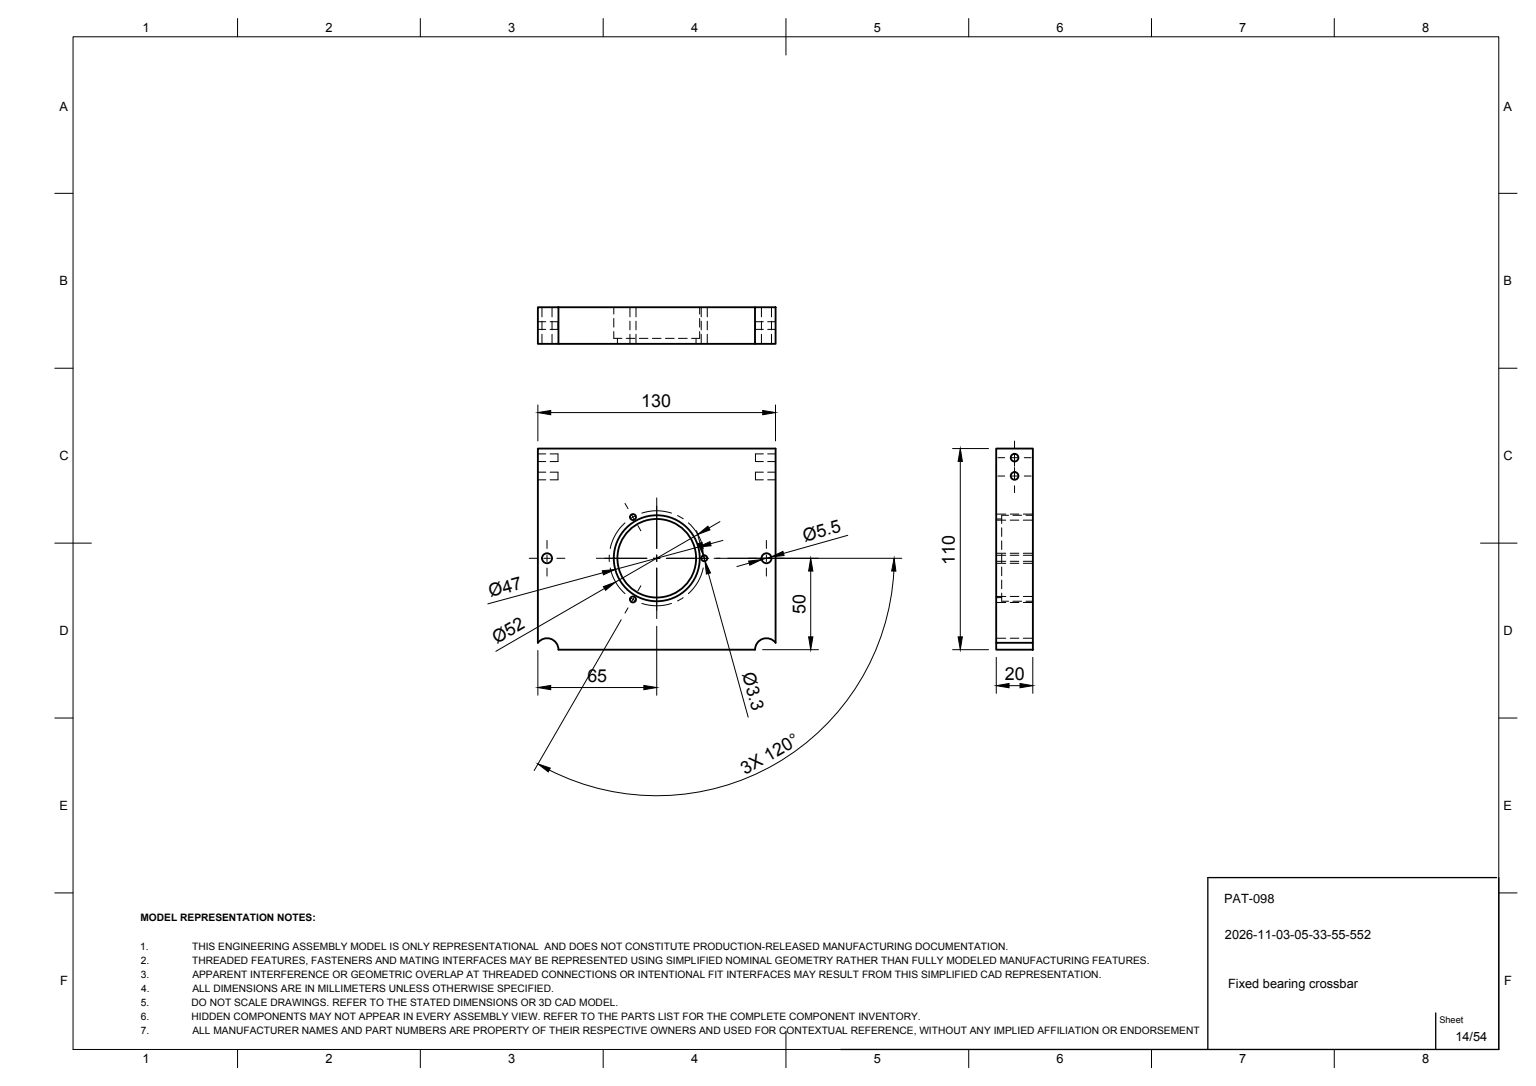
ISO-10303-21;
HEADER;
/* Generated by software containing ST-Developer
 * from STEP Tools, Inc. (www.steptools.com) 
 */

FILE_DESCRIPTION(
/* description */ ('Spring compression tester'),
/* implementation_level */ '2;1');

FILE_NAME(
/* name */ 'Fixed bearing crossbar.step',
/* time_stamp */ '2026-10-28T03:24:11-07:00',
/* author */ (''),
/* organization */ (''),
/* preprocessor_version */ 'ST-DEVELOPER v20.2',
/* originating_system */ 'Autodesk Translation Framework v15.17.0.0',
/* authorisation */ '');

FILE_SCHEMA (('AUTOMOTIVE_DESIGN { 1 0 10303 214 3 1 1 }'));
ENDSEC;

DATA;
#10=MECHANICAL_DESIGN_GEOMETRIC_PRESENTATION_REPRESENTATION('',(#1115),#43521);
#995=SHAPE_REPRESENTATION_RELATIONSHIP('SRR','None',#43807,#1055);
#1055=ADVANCED_BREP_SHAPE_REPRESENTATION('',(#1190),#43467);
#1115=STYLED_ITEM('',(#44202),#1190);
#1190=MANIFOLD_SOLID_BREP('Body1',#18552);
#1359=FACE_BOUND('',#3516,.T.);
#1360=FACE_BOUND('',#3521,.T.);
#1361=FACE_BOUND('',#3522,.T.);
#1362=FACE_BOUND('',#3524,.T.);
#1363=FACE_BOUND('',#3525,.T.);
#1364=FACE_BOUND('',#3526,.T.);
#1365=FACE_BOUND('',#3527,.T.);
#1366=FACE_BOUND('',#3528,.T.);
#1367=FACE_BOUND('',#3529,.T.);
#1368=FACE_BOUND('',#3533,.T.);
#1369=FACE_BOUND('',#3534,.T.);
#1370=FACE_BOUND('',#3536,.T.);
#1371=FACE_BOUND('',#3537,.T.);
#1372=FACE_BOUND('',#3538,.T.);
#1373=FACE_BOUND('',#3539,.T.);
#1374=FACE_BOUND('',#3540,.T.);
#1375=FACE_BOUND('',#3541,.T.);
#1693=PLANE('',#19632);
#1694=PLANE('',#19636);
#1695=PLANE('',#19640);
#1696=PLANE('',#19644);
#1697=PLANE('',#19648);
#1698=PLANE('',#19658);
#1699=PLANE('',#19659);
#1700=PLANE('',#19660);
#1701=PLANE('',#19661);
#1702=PLANE('',#19662);
#1703=PLANE('',#19663);
#2342=FACE_OUTER_BOUND('',#3501,.T.);
#2343=FACE_OUTER_BOUND('',#3502,.T.);
#2344=FACE_OUTER_BOUND('',#3503,.T.);
#2345=FACE_OUTER_BOUND('',#3504,.T.);
#2346=FACE_OUTER_BOUND('',#3505,.T.);
#2347=FACE_OUTER_BOUND('',#3506,.T.);
#2348=FACE_OUTER_BOUND('',#3507,.T.);
#2349=FACE_OUTER_BOUND('',#3508,.T.);
#2350=FACE_OUTER_BOUND('',#3509,.T.);
#2351=FACE_OUTER_BOUND('',#3510,.T.);
#2352=FACE_OUTER_BOUND('',#3511,.T.);
#2353=FACE_OUTER_BOUND('',#3512,.T.);
#2354=FACE_OUTER_BOUND('',#3513,.T.);
#2355=FACE_OUTER_BOUND('',#3514,.T.);
#2356=FACE_OUTER_BOUND('',#3515,.T.);
#2357=FACE_OUTER_BOUND('',#3517,.T.);
#2358=FACE_OUTER_BOUND('',#3518,.T.);
#2359=FACE_OUTER_BOUND('',#3519,.T.);
#2360=FACE_OUTER_BOUND('',#3520,.T.);
#2361=FACE_OUTER_BOUND('',#3523,.T.);
#2362=FACE_OUTER_BOUND('',#3530,.T.);
#2363=FACE_OUTER_BOUND('',#3531,.T.);
#2364=FACE_OUTER_BOUND('',#3532,.T.);
#2365=FACE_OUTER_BOUND('',#3535,.T.);
#3501=EDGE_LOOP('',(#13009,#13010,#13011,#13012));
#3502=EDGE_LOOP('',(#13013,#13014,#13015,#13016));
#3503=EDGE_LOOP('',(#13017,#13018,#13019,#13020));
#3504=EDGE_LOOP('',(#13021,#13022,#13023,#13024));
#3505=EDGE_LOOP('',(#13025,#13026,#13027,#13028));
#3506=EDGE_LOOP('',(#13029,#13030,#13031,#13032));
#3507=EDGE_LOOP('',(#13033));
#3508=EDGE_LOOP('',(#13034,#13035,#13036,#13037));
#3509=EDGE_LOOP('',(#13038));
#3510=EDGE_LOOP('',(#13039,#13040,#13041,#13042));
#3511=EDGE_LOOP('',(#13043));
#3512=EDGE_LOOP('',(#13044,#13045,#13046,#13047));
#3513=EDGE_LOOP('',(#13048));
#3514=EDGE_LOOP('',(#13049,#13050,#13051,#13052));
#3515=EDGE_LOOP('',(#13053));
#3516=EDGE_LOOP('',(#13054));
#3517=EDGE_LOOP('',(#13055,#13056,#13057,#13058));
#3518=EDGE_LOOP('',(#13059,#13060,#13061,#13062));
#3519=EDGE_LOOP('',(#13063,#13064,#13065,#13066));
#3520=EDGE_LOOP('',(#13067,#13068,#13069,#13070));
#3521=EDGE_LOOP('',(#13071));
#3522=EDGE_LOOP('',(#13072));
#3523=EDGE_LOOP('',(#13073,#13074,#13075,#13076,#13077,#13078));
#3524=EDGE_LOOP('',(#13079));
#3525=EDGE_LOOP('',(#13080));
#3526=EDGE_LOOP('',(#13081));
#3527=EDGE_LOOP('',(#13082));
#3528=EDGE_LOOP('',(#13083));
#3529=EDGE_LOOP('',(#13084));
#3530=EDGE_LOOP('',(#13085,#13086,#13087,#13088));
#3531=EDGE_LOOP('',(#13089,#13090,#13091,#13092));
#3532=EDGE_LOOP('',(#13093,#13094,#13095,#13096));
#3533=EDGE_LOOP('',(#13097));
#3534=EDGE_LOOP('',(#13098));
#3535=EDGE_LOOP('',(#13099,#13100,#13101,#13102,#13103,#13104));
#3536=EDGE_LOOP('',(#13105));
#3537=EDGE_LOOP('',(#13106));
#3538=EDGE_LOOP('',(#13107));
#3539=EDGE_LOOP('',(#13108));
#3540=EDGE_LOOP('',(#13109));
#3541=EDGE_LOOP('',(#13110));
#4858=LINE('',#27302,#6290);
#4859=LINE('',#27308,#6291);
#4860=LINE('',#27314,#6292);
#4861=LINE('',#27320,#6293);
#4862=LINE('',#27326,#6294);
#4863=LINE('',#27332,#6295);
#4864=LINE('',#27339,#6296);
#4865=LINE('',#27346,#6297);
#4866=LINE('',#27353,#6298);
#4867=LINE('',#27360,#6299);
#4868=LINE('',#27368,#6300);
#4869=LINE('',#27372,#6301);
#4870=LINE('',#27376,#6302);
#4871=LINE('',#27381,#6303);
#4872=LINE('',#27385,#6304);
#4873=LINE('',#27389,#6305);
#4874=LINE('',#27391,#6306);
#4875=LINE('',#27392,#6307);
#4876=LINE('',#27395,#6308);
#4877=LINE('',#27396,#6309);
#4878=LINE('',#27397,#6310);
#4879=LINE('',#27399,#6311);
#4880=LINE('',#27402,#6312);
#4881=LINE('',#27403,#6313);
#4882=LINE('',#27405,#6314);
#6290=VECTOR('',#22112,0.275);
#6291=VECTOR('',#22119,0.275);
#6292=VECTOR('',#22126,0.165);
#6293=VECTOR('',#22133,0.165);
#6294=VECTOR('',#22140,0.165);
#6295=VECTOR('',#22147,0.210000000000001);
#6296=VECTOR('',#22156,0.210000000000001);
#6297=VECTOR('',#22165,0.210000000000001);
#6298=VECTOR('',#22174,0.210000000000001);
#6299=VECTOR('',#22183,2.35);
#6300=VECTOR('',#22194,2.15);
#6301=VECTOR('',#22197,1.);
#6302=VECTOR('',#22200,1.);
#6303=VECTOR('',#22205,1.);
#6304=VECTOR('',#22208,1.);
#6305=VECTOR('',#22213,1.);
#6306=VECTOR('',#22214,1.);
#6307=VECTOR('',#22215,1.);
#6308=VECTOR('',#22218,1.);
#6309=VECTOR('',#22219,1.);
#6310=VECTOR('',#22220,1.);
#6311=VECTOR('',#22223,1.);
#6312=VECTOR('',#22226,1.);
#6313=VECTOR('',#22227,1.);
#6314=VECTOR('',#22230,1.);
#7614=CIRCLE('',#19615,0.275);
#7615=CIRCLE('',#19616,0.275);
#7616=CIRCLE('',#19618,0.275);
#7617=CIRCLE('',#19619,0.275);
#7618=CIRCLE('',#19621,0.165);
#7619=CIRCLE('',#19622,0.165);
#7620=CIRCLE('',#19624,0.165);
#7621=CIRCLE('',#19625,0.165);
#7622=CIRCLE('',#19627,0.165);
#7623=CIRCLE('',#19628,0.165);
#7624=CIRCLE('',#19630,0.210000000000001);
#7625=CIRCLE('',#19631,0.210000000000001);
#7626=CIRCLE('',#19634,0.210000000000001);
#7627=CIRCLE('',#19635,0.210000000000001);
#7628=CIRCLE('',#19638,0.210000000000001);
#7629=CIRCLE('',#19639,0.210000000000001);
#7630=CIRCLE('',#19642,0.210000000000001);
#7631=CIRCLE('',#19643,0.210000000000001);
#7632=CIRCLE('',#19646,2.35);
#7633=CIRCLE('',#19647,2.35);
#7634=CIRCLE('',#19649,2.15);
#7635=CIRCLE('',#19651,2.15);
#7636=CIRCLE('',#19653,0.625);
#7637=CIRCLE('',#19654,0.625);
#7638=CIRCLE('',#19656,0.625);
#7639=CIRCLE('',#19657,0.625);
#8400=VERTEX_POINT('',#27299);
#8401=VERTEX_POINT('',#27301);
#8402=VERTEX_POINT('',#27305);
#8403=VERTEX_POINT('',#27307);
#8404=VERTEX_POINT('',#27311);
#8405=VERTEX_POINT('',#27313);
#8406=VERTEX_POINT('',#27317);
#8407=VERTEX_POINT('',#27319);
#8408=VERTEX_POINT('',#27323);
#8409=VERTEX_POINT('',#27325);
#8410=VERTEX_POINT('',#27329);
#8411=VERTEX_POINT('',#27331);
#8412=VERTEX_POINT('',#27336);
#8413=VERTEX_POINT('',#27338);
#8414=VERTEX_POINT('',#27343);
#8415=VERTEX_POINT('',#27345);
#8416=VERTEX_POINT('',#27350);
#8417=VERTEX_POINT('',#27352);
#8418=VERTEX_POINT('',#27357);
#8419=VERTEX_POINT('',#27359);
#8420=VERTEX_POINT('',#27363);
#8421=VERTEX_POINT('',#27366);
#8422=VERTEX_POINT('',#27370);
#8423=VERTEX_POINT('',#27371);
#8424=VERTEX_POINT('',#27373);
#8425=VERTEX_POINT('',#27375);
#8426=VERTEX_POINT('',#27379);
#8427=VERTEX_POINT('',#27380);
#8428=VERTEX_POINT('',#27382);
#8429=VERTEX_POINT('',#27384);
#8430=VERTEX_POINT('',#27388);
#8431=VERTEX_POINT('',#27390);
#8432=VERTEX_POINT('',#27394);
#8433=VERTEX_POINT('',#27401);
#10169=EDGE_CURVE('',#8400,#8400,#7614,.T.);
#10170=EDGE_CURVE('',#8400,#8401,#4858,.T.);
#10171=EDGE_CURVE('',#8401,#8401,#7615,.T.);
#10172=EDGE_CURVE('',#8402,#8402,#7616,.T.);
#10173=EDGE_CURVE('',#8402,#8403,#4859,.T.);
#10174=EDGE_CURVE('',#8403,#8403,#7617,.T.);
#10175=EDGE_CURVE('',#8404,#8404,#7618,.T.);
#10176=EDGE_CURVE('',#8404,#8405,#4860,.T.);
#10177=EDGE_CURVE('',#8405,#8405,#7619,.T.);
#10178=EDGE_CURVE('',#8406,#8406,#7620,.T.);
#10179=EDGE_CURVE('',#8406,#8407,#4861,.T.);
#10180=EDGE_CURVE('',#8407,#8407,#7621,.T.);
#10181=EDGE_CURVE('',#8408,#8408,#7622,.T.);
#10182=EDGE_CURVE('',#8408,#8409,#4862,.T.);
#10183=EDGE_CURVE('',#8409,#8409,#7623,.T.);
#10184=EDGE_CURVE('',#8410,#8410,#7624,.T.);
#10185=EDGE_CURVE('',#8410,#8411,#4863,.T.);
#10186=EDGE_CURVE('',#8411,#8411,#7625,.T.);
#10187=EDGE_CURVE('',#8412,#8412,#7626,.T.);
#10188=EDGE_CURVE('',#8412,#8413,#4864,.T.);
#10189=EDGE_CURVE('',#8413,#8413,#7627,.T.);
#10190=EDGE_CURVE('',#8414,#8414,#7628,.T.);
#10191=EDGE_CURVE('',#8414,#8415,#4865,.T.);
#10192=EDGE_CURVE('',#8415,#8415,#7629,.T.);
#10193=EDGE_CURVE('',#8416,#8416,#7630,.T.);
#10194=EDGE_CURVE('',#8416,#8417,#4866,.T.);
#10195=EDGE_CURVE('',#8417,#8417,#7631,.T.);
#10196=EDGE_CURVE('',#8418,#8418,#7632,.T.);
#10197=EDGE_CURVE('',#8418,#8419,#4867,.T.);
#10198=EDGE_CURVE('',#8419,#8419,#7633,.T.);
#10199=EDGE_CURVE('',#8420,#8420,#7634,.T.);
#10200=EDGE_CURVE('',#8421,#8421,#7635,.T.);
#10201=EDGE_CURVE('',#8421,#8420,#4868,.T.);
#10202=EDGE_CURVE('',#8422,#8423,#4869,.T.);
#10203=EDGE_CURVE('',#8424,#8422,#7636,.T.);
#10204=EDGE_CURVE('',#8425,#8424,#4870,.T.);
#10205=EDGE_CURVE('',#8423,#8425,#7637,.T.);
#10206=EDGE_CURVE('',#8426,#8427,#4871,.T.);
#10207=EDGE_CURVE('',#8428,#8426,#7638,.T.);
#10208=EDGE_CURVE('',#8429,#8428,#4872,.T.);
#10209=EDGE_CURVE('',#8427,#8429,#7639,.T.);
#10210=EDGE_CURVE('',#8428,#8430,#4873,.T.);
#10211=EDGE_CURVE('',#8430,#8431,#4874,.T.);
#10212=EDGE_CURVE('',#8429,#8431,#4875,.T.);
#10213=EDGE_CURVE('',#8432,#8422,#4876,.T.);
#10214=EDGE_CURVE('',#8430,#8432,#4877,.T.);
#10215=EDGE_CURVE('',#8424,#8426,#4878,.T.);
#10216=EDGE_CURVE('',#8425,#8427,#4879,.T.);
#10217=EDGE_CURVE('',#8432,#8433,#4880,.T.);
#10218=EDGE_CURVE('',#8431,#8433,#4881,.T.);
#10219=EDGE_CURVE('',#8433,#8423,#4882,.T.);
#13009=ORIENTED_EDGE('',*,*,#10169,.F.);
#13010=ORIENTED_EDGE('',*,*,#10170,.T.);
#13011=ORIENTED_EDGE('',*,*,#10171,.F.);
#13012=ORIENTED_EDGE('',*,*,#10170,.F.);
#13013=ORIENTED_EDGE('',*,*,#10172,.F.);
#13014=ORIENTED_EDGE('',*,*,#10173,.T.);
#13015=ORIENTED_EDGE('',*,*,#10174,.F.);
#13016=ORIENTED_EDGE('',*,*,#10173,.F.);
#13017=ORIENTED_EDGE('',*,*,#10175,.F.);
#13018=ORIENTED_EDGE('',*,*,#10176,.T.);
#13019=ORIENTED_EDGE('',*,*,#10177,.F.);
#13020=ORIENTED_EDGE('',*,*,#10176,.F.);
#13021=ORIENTED_EDGE('',*,*,#10178,.F.);
#13022=ORIENTED_EDGE('',*,*,#10179,.T.);
#13023=ORIENTED_EDGE('',*,*,#10180,.F.);
#13024=ORIENTED_EDGE('',*,*,#10179,.F.);
#13025=ORIENTED_EDGE('',*,*,#10181,.F.);
#13026=ORIENTED_EDGE('',*,*,#10182,.T.);
#13027=ORIENTED_EDGE('',*,*,#10183,.F.);
#13028=ORIENTED_EDGE('',*,*,#10182,.F.);
#13029=ORIENTED_EDGE('',*,*,#10184,.F.);
#13030=ORIENTED_EDGE('',*,*,#10185,.T.);
#13031=ORIENTED_EDGE('',*,*,#10186,.F.);
#13032=ORIENTED_EDGE('',*,*,#10185,.F.);
#13033=ORIENTED_EDGE('',*,*,#10184,.T.);
#13034=ORIENTED_EDGE('',*,*,#10187,.F.);
#13035=ORIENTED_EDGE('',*,*,#10188,.T.);
#13036=ORIENTED_EDGE('',*,*,#10189,.F.);
#13037=ORIENTED_EDGE('',*,*,#10188,.F.);
#13038=ORIENTED_EDGE('',*,*,#10187,.T.);
#13039=ORIENTED_EDGE('',*,*,#10190,.F.);
#13040=ORIENTED_EDGE('',*,*,#10191,.T.);
#13041=ORIENTED_EDGE('',*,*,#10192,.T.);
#13042=ORIENTED_EDGE('',*,*,#10191,.F.);
#13043=ORIENTED_EDGE('',*,*,#10192,.F.);
#13044=ORIENTED_EDGE('',*,*,#10193,.F.);
#13045=ORIENTED_EDGE('',*,*,#10194,.T.);
#13046=ORIENTED_EDGE('',*,*,#10195,.T.);
#13047=ORIENTED_EDGE('',*,*,#10194,.F.);
#13048=ORIENTED_EDGE('',*,*,#10195,.F.);
#13049=ORIENTED_EDGE('',*,*,#10196,.F.);
#13050=ORIENTED_EDGE('',*,*,#10197,.T.);
#13051=ORIENTED_EDGE('',*,*,#10198,.F.);
#13052=ORIENTED_EDGE('',*,*,#10197,.F.);
#13053=ORIENTED_EDGE('',*,*,#10196,.T.);
#13054=ORIENTED_EDGE('',*,*,#10199,.F.);
#13055=ORIENTED_EDGE('',*,*,#10200,.F.);
#13056=ORIENTED_EDGE('',*,*,#10201,.T.);
#13057=ORIENTED_EDGE('',*,*,#10199,.T.);
#13058=ORIENTED_EDGE('',*,*,#10201,.F.);
#13059=ORIENTED_EDGE('',*,*,#10202,.F.);
#13060=ORIENTED_EDGE('',*,*,#10203,.F.);
#13061=ORIENTED_EDGE('',*,*,#10204,.F.);
#13062=ORIENTED_EDGE('',*,*,#10205,.F.);
#13063=ORIENTED_EDGE('',*,*,#10206,.F.);
#13064=ORIENTED_EDGE('',*,*,#10207,.F.);
#13065=ORIENTED_EDGE('',*,*,#10208,.F.);
#13066=ORIENTED_EDGE('',*,*,#10209,.F.);
#13067=ORIENTED_EDGE('',*,*,#10208,.T.);
#13068=ORIENTED_EDGE('',*,*,#10210,.T.);
#13069=ORIENTED_EDGE('',*,*,#10211,.T.);
#13070=ORIENTED_EDGE('',*,*,#10212,.F.);
#13071=ORIENTED_EDGE('',*,*,#10186,.T.);
#13072=ORIENTED_EDGE('',*,*,#10189,.T.);
#13073=ORIENTED_EDGE('',*,*,#10203,.T.);
#13074=ORIENTED_EDGE('',*,*,#10213,.F.);
#13075=ORIENTED_EDGE('',*,*,#10214,.F.);
#13076=ORIENTED_EDGE('',*,*,#10210,.F.);
#13077=ORIENTED_EDGE('',*,*,#10207,.T.);
#13078=ORIENTED_EDGE('',*,*,#10215,.F.);
#13079=ORIENTED_EDGE('',*,*,#10169,.T.);
#13080=ORIENTED_EDGE('',*,*,#10172,.T.);
#13081=ORIENTED_EDGE('',*,*,#10175,.T.);
#13082=ORIENTED_EDGE('',*,*,#10178,.T.);
#13083=ORIENTED_EDGE('',*,*,#10181,.T.);
#13084=ORIENTED_EDGE('',*,*,#10200,.T.);
#13085=ORIENTED_EDGE('',*,*,#10204,.T.);
#13086=ORIENTED_EDGE('',*,*,#10215,.T.);
#13087=ORIENTED_EDGE('',*,*,#10206,.T.);
#13088=ORIENTED_EDGE('',*,*,#10216,.F.);
#13089=ORIENTED_EDGE('',*,*,#10214,.T.);
#13090=ORIENTED_EDGE('',*,*,#10217,.T.);
#13091=ORIENTED_EDGE('',*,*,#10218,.F.);
#13092=ORIENTED_EDGE('',*,*,#10211,.F.);
#13093=ORIENTED_EDGE('',*,*,#10202,.T.);
#13094=ORIENTED_EDGE('',*,*,#10219,.F.);
#13095=ORIENTED_EDGE('',*,*,#10217,.F.);
#13096=ORIENTED_EDGE('',*,*,#10213,.T.);
#13097=ORIENTED_EDGE('',*,*,#10190,.T.);
#13098=ORIENTED_EDGE('',*,*,#10193,.T.);
#13099=ORIENTED_EDGE('',*,*,#10205,.T.);
#13100=ORIENTED_EDGE('',*,*,#10216,.T.);
#13101=ORIENTED_EDGE('',*,*,#10209,.T.);
#13102=ORIENTED_EDGE('',*,*,#10212,.T.);
#13103=ORIENTED_EDGE('',*,*,#10218,.T.);
#13104=ORIENTED_EDGE('',*,*,#10219,.T.);
#13105=ORIENTED_EDGE('',*,*,#10171,.T.);
#13106=ORIENTED_EDGE('',*,*,#10174,.T.);
#13107=ORIENTED_EDGE('',*,*,#10177,.T.);
#13108=ORIENTED_EDGE('',*,*,#10180,.T.);
#13109=ORIENTED_EDGE('',*,*,#10183,.T.);
#13110=ORIENTED_EDGE('',*,*,#10198,.T.);
#17173=CYLINDRICAL_SURFACE('',#19614,0.275);
#17174=CYLINDRICAL_SURFACE('',#19617,0.275);
#17175=CYLINDRICAL_SURFACE('',#19620,0.165);
#17176=CYLINDRICAL_SURFACE('',#19623,0.165);
#17177=CYLINDRICAL_SURFACE('',#19626,0.165);
#17178=CYLINDRICAL_SURFACE('',#19629,0.210000000000001);
#17179=CYLINDRICAL_SURFACE('',#19633,0.210000000000001);
#17180=CYLINDRICAL_SURFACE('',#19637,0.210000000000001);
#17181=CYLINDRICAL_SURFACE('',#19641,0.210000000000001);
#17182=CYLINDRICAL_SURFACE('',#19645,2.35);
#17183=CYLINDRICAL_SURFACE('',#19650,2.15);
#17184=CYLINDRICAL_SURFACE('',#19652,0.625);
#17185=CYLINDRICAL_SURFACE('',#19655,0.625);
#17666=ADVANCED_FACE('',(#2342),#17173,.F.);
#17667=ADVANCED_FACE('',(#2343),#17174,.F.);
#17668=ADVANCED_FACE('',(#2344),#17175,.F.);
#17669=ADVANCED_FACE('',(#2345),#17176,.F.);
#17670=ADVANCED_FACE('',(#2346),#17177,.F.);
#17671=ADVANCED_FACE('',(#2347),#17178,.F.);
#17672=ADVANCED_FACE('',(#2348),#1693,.T.);
#17673=ADVANCED_FACE('',(#2349),#17179,.F.);
#17674=ADVANCED_FACE('',(#2350),#1694,.T.);
#17675=ADVANCED_FACE('',(#2351),#17180,.F.);
#17676=ADVANCED_FACE('',(#2352),#1695,.F.);
#17677=ADVANCED_FACE('',(#2353),#17181,.F.);
#17678=ADVANCED_FACE('',(#2354),#1696,.F.);
#17679=ADVANCED_FACE('',(#2355),#17182,.F.);
#17680=ADVANCED_FACE('',(#2356,#1359),#1697,.T.);
#17681=ADVANCED_FACE('',(#2357),#17183,.F.);
#17682=ADVANCED_FACE('',(#2358),#17184,.F.);
#17683=ADVANCED_FACE('',(#2359),#17185,.F.);
#17684=ADVANCED_FACE('',(#2360,#1360,#1361),#1698,.T.);
#17685=ADVANCED_FACE('',(#2361,#1362,#1363,#1364,#1365,#1366,#1367),#1699,
 .F.);
#17686=ADVANCED_FACE('',(#2362),#1700,.T.);
#17687=ADVANCED_FACE('',(#2363),#1701,.T.);
#17688=ADVANCED_FACE('',(#2364,#1368,#1369),#1702,.T.);
#17689=ADVANCED_FACE('',(#2365,#1370,#1371,#1372,#1373,#1374,#1375),#1703,
 .T.);
#18552=CLOSED_SHELL('',(#17666,#17667,#17668,#17669,#17670,#17671,#17672,
#17673,#17674,#17675,#17676,#17677,#17678,#17679,#17680,#17681,#17682,#17683,
#17684,#17685,#17686,#17687,#17688,#17689));
#19613=AXIS2_PLACEMENT_3D('',#27297,#22106,#22107);
#19614=AXIS2_PLACEMENT_3D('',#27298,#22108,#22109);
#19615=AXIS2_PLACEMENT_3D('',#27300,#22110,#22111);
#19616=AXIS2_PLACEMENT_3D('',#27303,#22113,#22114);
#19617=AXIS2_PLACEMENT_3D('',#27304,#22115,#22116);
#19618=AXIS2_PLACEMENT_3D('',#27306,#22117,#22118);
#19619=AXIS2_PLACEMENT_3D('',#27309,#22120,#22121);
#19620=AXIS2_PLACEMENT_3D('',#27310,#22122,#22123);
#19621=AXIS2_PLACEMENT_3D('',#27312,#22124,#22125);
#19622=AXIS2_PLACEMENT_3D('',#27315,#22127,#22128);
#19623=AXIS2_PLACEMENT_3D('',#27316,#22129,#22130);
#19624=AXIS2_PLACEMENT_3D('',#27318,#22131,#22132);
#19625=AXIS2_PLACEMENT_3D('',#27321,#22134,#22135);
#19626=AXIS2_PLACEMENT_3D('',#27322,#22136,#22137);
#19627=AXIS2_PLACEMENT_3D('',#27324,#22138,#22139);
#19628=AXIS2_PLACEMENT_3D('',#27327,#22141,#22142);
#19629=AXIS2_PLACEMENT_3D('',#27328,#22143,#22144);
#19630=AXIS2_PLACEMENT_3D('',#27330,#22145,#22146);
#19631=AXIS2_PLACEMENT_3D('',#27333,#22148,#22149);
#19632=AXIS2_PLACEMENT_3D('',#27334,#22150,#22151);
#19633=AXIS2_PLACEMENT_3D('',#27335,#22152,#22153);
#19634=AXIS2_PLACEMENT_3D('',#27337,#22154,#22155);
#19635=AXIS2_PLACEMENT_3D('',#27340,#22157,#22158);
#19636=AXIS2_PLACEMENT_3D('',#27341,#22159,#22160);
#19637=AXIS2_PLACEMENT_3D('',#27342,#22161,#22162);
#19638=AXIS2_PLACEMENT_3D('',#27344,#22163,#22164);
#19639=AXIS2_PLACEMENT_3D('',#27347,#22166,#22167);
#19640=AXIS2_PLACEMENT_3D('',#27348,#22168,#22169);
#19641=AXIS2_PLACEMENT_3D('',#27349,#22170,#22171);
#19642=AXIS2_PLACEMENT_3D('',#27351,#22172,#22173);
#19643=AXIS2_PLACEMENT_3D('',#27354,#22175,#22176);
#19644=AXIS2_PLACEMENT_3D('',#27355,#22177,#22178);
#19645=AXIS2_PLACEMENT_3D('',#27356,#22179,#22180);
#19646=AXIS2_PLACEMENT_3D('',#27358,#22181,#22182);
#19647=AXIS2_PLACEMENT_3D('',#27361,#22184,#22185);
#19648=AXIS2_PLACEMENT_3D('',#27362,#22186,#22187);
#19649=AXIS2_PLACEMENT_3D('',#27364,#22188,#22189);
#19650=AXIS2_PLACEMENT_3D('',#27365,#22190,#22191);
#19651=AXIS2_PLACEMENT_3D('',#27367,#22192,#22193);
#19652=AXIS2_PLACEMENT_3D('',#27369,#22195,#22196);
#19653=AXIS2_PLACEMENT_3D('',#27374,#22198,#22199);
#19654=AXIS2_PLACEMENT_3D('',#27377,#22201,#22202);
#19655=AXIS2_PLACEMENT_3D('',#27378,#22203,#22204);
#19656=AXIS2_PLACEMENT_3D('',#27383,#22206,#22207);
#19657=AXIS2_PLACEMENT_3D('',#27386,#22209,#22210);
#19658=AXIS2_PLACEMENT_3D('',#27387,#22211,#22212);
#19659=AXIS2_PLACEMENT_3D('',#27393,#22216,#22217);
#19660=AXIS2_PLACEMENT_3D('',#27398,#22221,#22222);
#19661=AXIS2_PLACEMENT_3D('',#27400,#22224,#22225);
#19662=AXIS2_PLACEMENT_3D('',#27404,#22228,#22229);
#19663=AXIS2_PLACEMENT_3D('',#27406,#22231,#22232);
#22106=DIRECTION('axis',(0.,0.,1.));
#22107=DIRECTION('refdir',(1.,0.,0.));
#22108=DIRECTION('center_axis',(0.,0.,1.));
#22109=DIRECTION('ref_axis',(1.,0.,0.));
#22110=DIRECTION('center_axis',(0.,0.,1.));
#22111=DIRECTION('ref_axis',(1.,0.,0.));
#22112=DIRECTION('',(0.,0.,1.));
#22113=DIRECTION('center_axis',(0.,0.,-1.));
#22114=DIRECTION('ref_axis',(1.,0.,0.));
#22115=DIRECTION('center_axis',(0.,0.,1.));
#22116=DIRECTION('ref_axis',(1.,0.,0.));
#22117=DIRECTION('center_axis',(0.,0.,1.));
#22118=DIRECTION('ref_axis',(1.,0.,0.));
#22119=DIRECTION('',(0.,0.,1.));
#22120=DIRECTION('center_axis',(0.,0.,-1.));
#22121=DIRECTION('ref_axis',(1.,0.,0.));
#22122=DIRECTION('center_axis',(0.,0.,1.));
#22123=DIRECTION('ref_axis',(1.,0.,0.));
#22124=DIRECTION('center_axis',(0.,0.,1.));
#22125=DIRECTION('ref_axis',(1.,0.,0.));
#22126=DIRECTION('',(0.,0.,1.));
#22127=DIRECTION('center_axis',(0.,0.,-1.));
#22128=DIRECTION('ref_axis',(1.,0.,0.));
#22129=DIRECTION('center_axis',(0.,0.,1.));
#22130=DIRECTION('ref_axis',(1.,0.,0.));
#22131=DIRECTION('center_axis',(0.,0.,1.));
#22132=DIRECTION('ref_axis',(1.,0.,0.));
#22133=DIRECTION('',(0.,0.,1.));
#22134=DIRECTION('center_axis',(0.,0.,-1.));
#22135=DIRECTION('ref_axis',(1.,0.,0.));
#22136=DIRECTION('center_axis',(0.,0.,1.));
#22137=DIRECTION('ref_axis',(1.,0.,0.));
#22138=DIRECTION('center_axis',(0.,0.,1.));
#22139=DIRECTION('ref_axis',(1.,0.,0.));
#22140=DIRECTION('',(0.,0.,1.));
#22141=DIRECTION('center_axis',(0.,0.,-1.));
#22142=DIRECTION('ref_axis',(1.,0.,0.));
#22143=DIRECTION('center_axis',(1.,0.,0.));
#22144=DIRECTION('ref_axis',(0.,0.,-1.));
#22145=DIRECTION('center_axis',(1.,0.,0.));
#22146=DIRECTION('ref_axis',(0.,0.,-1.));
#22147=DIRECTION('',(1.,0.,0.));
#22148=DIRECTION('center_axis',(-1.,0.,0.));
#22149=DIRECTION('ref_axis',(0.,0.,-1.));
#22150=DIRECTION('center_axis',(1.,0.,0.));
#22151=DIRECTION('ref_axis',(0.,0.,-1.));
#22152=DIRECTION('center_axis',(1.,0.,0.));
#22153=DIRECTION('ref_axis',(0.,0.,-1.));
#22154=DIRECTION('center_axis',(1.,0.,0.));
#22155=DIRECTION('ref_axis',(0.,0.,-1.));
#22156=DIRECTION('',(1.,0.,0.));
#22157=DIRECTION('center_axis',(-1.,0.,0.));
#22158=DIRECTION('ref_axis',(0.,0.,-1.));
#22159=DIRECTION('center_axis',(1.,0.,0.));
#22160=DIRECTION('ref_axis',(0.,0.,-1.));
#22161=DIRECTION('center_axis',(1.,0.,0.));
#22162=DIRECTION('ref_axis',(0.,0.,-1.));
#22163=DIRECTION('center_axis',(1.,0.,0.));
#22164=DIRECTION('ref_axis',(0.,0.,-1.));
#22165=DIRECTION('',(1.,0.,0.));
#22166=DIRECTION('center_axis',(1.,0.,0.));
#22167=DIRECTION('ref_axis',(0.,0.,-1.));
#22168=DIRECTION('center_axis',(1.,0.,0.));
#22169=DIRECTION('ref_axis',(0.,0.,-1.));
#22170=DIRECTION('center_axis',(1.,0.,0.));
#22171=DIRECTION('ref_axis',(0.,0.,-1.));
#22172=DIRECTION('center_axis',(1.,0.,0.));
#22173=DIRECTION('ref_axis',(0.,0.,-1.));
#22174=DIRECTION('',(1.,0.,0.));
#22175=DIRECTION('center_axis',(1.,0.,0.));
#22176=DIRECTION('ref_axis',(0.,0.,-1.));
#22177=DIRECTION('center_axis',(1.,0.,0.));
#22178=DIRECTION('ref_axis',(0.,0.,-1.));
#22179=DIRECTION('center_axis',(0.,0.,1.));
#22180=DIRECTION('ref_axis',(1.,0.,0.));
#22181=DIRECTION('center_axis',(0.,0.,1.));
#22182=DIRECTION('ref_axis',(1.,0.,0.));
#22183=DIRECTION('',(0.,0.,1.));
#22184=DIRECTION('center_axis',(0.,0.,-1.));
#22185=DIRECTION('ref_axis',(1.,0.,0.));
#22186=DIRECTION('center_axis',(0.,0.,1.));
#22187=DIRECTION('ref_axis',(1.,0.,0.));
#22188=DIRECTION('center_axis',(0.,0.,1.));
#22189=DIRECTION('ref_axis',(1.,0.,0.));
#22190=DIRECTION('center_axis',(0.,0.,1.));
#22191=DIRECTION('ref_axis',(1.,0.,0.));
#22192=DIRECTION('center_axis',(0.,0.,1.));
#22193=DIRECTION('ref_axis',(1.,0.,0.));
#22194=DIRECTION('',(0.,0.,1.));
#22195=DIRECTION('center_axis',(0.,0.,1.));
#22196=DIRECTION('ref_axis',(1.,0.,0.));
#22197=DIRECTION('',(0.,0.,1.));
#22198=DIRECTION('center_axis',(0.,0.,1.));
#22199=DIRECTION('ref_axis',(1.,0.,0.));
#22200=DIRECTION('',(0.,0.,-1.));
#22201=DIRECTION('center_axis',(0.,0.,-1.));
#22202=DIRECTION('ref_axis',(1.,0.,0.));
#22203=DIRECTION('center_axis',(0.,0.,1.));
#22204=DIRECTION('ref_axis',(1.,0.,0.));
#22205=DIRECTION('',(0.,0.,1.));
#22206=DIRECTION('center_axis',(0.,0.,1.));
#22207=DIRECTION('ref_axis',(1.,0.,0.));
#22208=DIRECTION('',(0.,0.,-1.));
#22209=DIRECTION('center_axis',(0.,0.,-1.));
#22210=DIRECTION('ref_axis',(1.,0.,0.));
#22211=DIRECTION('center_axis',(1.,0.,0.));
#22212=DIRECTION('ref_axis',(0.,1.,0.));
#22213=DIRECTION('',(0.,1.,0.));
#22214=DIRECTION('',(0.,0.,1.));
#22215=DIRECTION('',(0.,1.,0.));
#22216=DIRECTION('center_axis',(0.,0.,1.));
#22217=DIRECTION('ref_axis',(1.,0.,0.));
#22218=DIRECTION('',(0.,-1.,0.));
#22219=DIRECTION('',(-1.,0.,0.));
#22220=DIRECTION('',(1.,0.,0.));
#22221=DIRECTION('center_axis',(0.,-1.,0.));
#22222=DIRECTION('ref_axis',(1.,0.,0.));
#22223=DIRECTION('',(1.,0.,0.));
#22224=DIRECTION('center_axis',(0.,1.,0.));
#22225=DIRECTION('ref_axis',(-1.,0.,0.));
#22226=DIRECTION('',(0.,0.,1.));
#22227=DIRECTION('',(-1.,0.,0.));
#22228=DIRECTION('center_axis',(-1.,0.,0.));
#22229=DIRECTION('ref_axis',(0.,-1.,0.));
#22230=DIRECTION('',(0.,-1.,0.));
#22231=DIRECTION('center_axis',(0.,0.,1.));
#22232=DIRECTION('ref_axis',(1.,0.,0.));
#27297=CARTESIAN_POINT('',(0.,0.,0.));
#27298=CARTESIAN_POINT('Origin',(6.,5.,22.9));
#27299=CARTESIAN_POINT('',(5.725,5.,23.));
#27300=CARTESIAN_POINT('Origin',(6.,5.,23.));
#27301=CARTESIAN_POINT('',(5.725,5.,25.));
#27302=CARTESIAN_POINT('',(5.725,5.,22.9));
#27303=CARTESIAN_POINT('Origin',(6.,5.,25.));
#27304=CARTESIAN_POINT('Origin',(-6.,5.,22.9));
#27305=CARTESIAN_POINT('',(-6.275,5.,23.));
#27306=CARTESIAN_POINT('Origin',(-6.,5.,23.));
#27307=CARTESIAN_POINT('',(-6.275,5.,25.));
#27308=CARTESIAN_POINT('',(-6.275,5.,22.9));
#27309=CARTESIAN_POINT('Origin',(-6.,5.,25.));
#27310=CARTESIAN_POINT('Origin',(2.6,5.,22.9));
#27311=CARTESIAN_POINT('',(2.435,5.,23.));
#27312=CARTESIAN_POINT('Origin',(2.6,5.,23.));
#27313=CARTESIAN_POINT('',(2.435,5.,25.));
#27314=CARTESIAN_POINT('',(2.435,5.,22.9));
#27315=CARTESIAN_POINT('Origin',(2.6,5.,25.));
#27316=CARTESIAN_POINT('Origin',(-1.3,7.25166604983954,22.9));
#27317=CARTESIAN_POINT('',(-1.465,7.25166604983954,23.));
#27318=CARTESIAN_POINT('Origin',(-1.3,7.25166604983954,23.));
#27319=CARTESIAN_POINT('',(-1.465,7.25166604983954,25.));
#27320=CARTESIAN_POINT('',(-1.465,7.25166604983954,22.9));
#27321=CARTESIAN_POINT('Origin',(-1.3,7.25166604983954,25.));
#27322=CARTESIAN_POINT('Origin',(-1.3,2.74833395016046,22.9));
#27323=CARTESIAN_POINT('',(-1.465,2.74833395016046,23.));
#27324=CARTESIAN_POINT('Origin',(-1.3,2.74833395016046,23.));
#27325=CARTESIAN_POINT('',(-1.465,2.74833395016046,25.));
#27326=CARTESIAN_POINT('',(-1.465,2.74833395016046,22.9));
#27327=CARTESIAN_POINT('Origin',(-1.3,2.74833395016046,25.));
#27328=CARTESIAN_POINT('Origin',(5.4,9.5,24.));
#27329=CARTESIAN_POINT('',(5.4,9.5,24.21));
#27330=CARTESIAN_POINT('Origin',(5.4,9.5,24.));
#27331=CARTESIAN_POINT('',(6.5,9.5,24.21));
#27332=CARTESIAN_POINT('',(5.4,9.5,24.21));
#27333=CARTESIAN_POINT('Origin',(6.5,9.5,24.));
#27334=CARTESIAN_POINT('Origin',(5.4,9.5,24.));
#27335=CARTESIAN_POINT('Origin',(5.4,10.5,24.));
#27336=CARTESIAN_POINT('',(5.4,10.5,24.21));
#27337=CARTESIAN_POINT('Origin',(5.4,10.5,24.));
#27338=CARTESIAN_POINT('',(6.5,10.5,24.21));
#27339=CARTESIAN_POINT('',(5.4,10.5,24.21));
#27340=CARTESIAN_POINT('Origin',(6.5,10.5,24.));
#27341=CARTESIAN_POINT('Origin',(5.4,10.5,24.));
#27342=CARTESIAN_POINT('Origin',(-6.6,9.5,24.));
#27343=CARTESIAN_POINT('',(-6.5,9.5,24.21));
#27344=CARTESIAN_POINT('Origin',(-6.5,9.5,24.));
#27345=CARTESIAN_POINT('',(-5.4,9.5,24.21));
#27346=CARTESIAN_POINT('',(-6.6,9.5,24.21));
#27347=CARTESIAN_POINT('Origin',(-5.4,9.5,24.));
#27348=CARTESIAN_POINT('Origin',(-5.4,9.5,24.));
#27349=CARTESIAN_POINT('Origin',(-6.6,10.5,24.));
#27350=CARTESIAN_POINT('',(-6.5,10.5,24.21));
#27351=CARTESIAN_POINT('Origin',(-6.5,10.5,24.));
#27352=CARTESIAN_POINT('',(-5.4,10.5,24.21));
#27353=CARTESIAN_POINT('',(-6.6,10.5,24.21));
#27354=CARTESIAN_POINT('Origin',(-5.4,10.5,24.));
#27355=CARTESIAN_POINT('Origin',(-5.4,10.5,24.));
#27356=CARTESIAN_POINT('Origin',(0.,5.,23.3));
#27357=CARTESIAN_POINT('',(-2.35,5.,23.3));
#27358=CARTESIAN_POINT('Origin',(0.,5.,23.3));
#27359=CARTESIAN_POINT('',(-2.35,5.,25.));
#27360=CARTESIAN_POINT('',(-2.35,5.,23.3));
#27361=CARTESIAN_POINT('Origin',(0.,5.,25.));
#27362=CARTESIAN_POINT('Origin',(0.,5.,23.3));
#27363=CARTESIAN_POINT('',(-2.15,5.,23.3));
#27364=CARTESIAN_POINT('Origin',(0.,5.,23.3));
#27365=CARTESIAN_POINT('Origin',(0.,5.,22.9));
#27366=CARTESIAN_POINT('',(-2.15,5.,23.));
#27367=CARTESIAN_POINT('Origin',(0.,5.,23.));
#27368=CARTESIAN_POINT('',(-2.15,5.,22.9));
#27369=CARTESIAN_POINT('Origin',(-6.,0.,22.9));
#27370=CARTESIAN_POINT('',(-6.5,0.375,23.));
#27371=CARTESIAN_POINT('',(-6.5,0.375,25.));
#27372=CARTESIAN_POINT('',(-6.5,0.375,22.9));
#27373=CARTESIAN_POINT('',(-5.375,0.,23.));
#27374=CARTESIAN_POINT('Origin',(-6.,0.,23.));
#27375=CARTESIAN_POINT('',(-5.375,0.,25.));
#27376=CARTESIAN_POINT('',(-5.375,0.,22.9));
#27377=CARTESIAN_POINT('Origin',(-6.,0.,25.));
#27378=CARTESIAN_POINT('Origin',(6.,0.,22.9));
#27379=CARTESIAN_POINT('',(5.375,0.,23.));
#27380=CARTESIAN_POINT('',(5.375,0.,25.));
#27381=CARTESIAN_POINT('',(5.375,0.,22.9));
#27382=CARTESIAN_POINT('',(6.5,0.375,23.));
#27383=CARTESIAN_POINT('Origin',(6.,0.,23.));
#27384=CARTESIAN_POINT('',(6.5,0.375,25.));
#27385=CARTESIAN_POINT('',(6.5,0.375,22.9));
#27386=CARTESIAN_POINT('Origin',(6.,0.,25.));
#27387=CARTESIAN_POINT('Origin',(6.5,0.,23.));
#27388=CARTESIAN_POINT('',(6.5,11.,23.));
#27389=CARTESIAN_POINT('',(6.5,0.,23.));
#27390=CARTESIAN_POINT('',(6.5,11.,25.));
#27391=CARTESIAN_POINT('',(6.5,11.,23.));
#27392=CARTESIAN_POINT('',(6.5,0.,25.));
#27393=CARTESIAN_POINT('Origin',(0.,5.5,23.));
#27394=CARTESIAN_POINT('',(-6.5,11.,23.));
#27395=CARTESIAN_POINT('',(-6.5,11.,23.));
#27396=CARTESIAN_POINT('',(6.5,11.,23.));
#27397=CARTESIAN_POINT('',(-6.5,0.,23.));
#27398=CARTESIAN_POINT('Origin',(-6.5,0.,23.));
#27399=CARTESIAN_POINT('',(-6.5,0.,25.));
#27400=CARTESIAN_POINT('Origin',(6.5,11.,23.));
#27401=CARTESIAN_POINT('',(-6.5,11.,25.));
#27402=CARTESIAN_POINT('',(-6.5,11.,23.));
#27403=CARTESIAN_POINT('',(6.5,11.,25.));
#27404=CARTESIAN_POINT('Origin',(-6.5,11.,23.));
#27405=CARTESIAN_POINT('',(-6.5,11.,25.));
#27406=CARTESIAN_POINT('Origin',(0.,5.5,25.));
#43399=UNCERTAINTY_MEASURE_WITH_UNIT(LENGTH_MEASURE(0.001),#43522,
'DISTANCE_ACCURACY_VALUE',
'Maximum model space distance between geometric entities at asserted c
onnectivities');
#43453=UNCERTAINTY_MEASURE_WITH_UNIT(LENGTH_MEASURE(0.001),#43522,
'DISTANCE_ACCURACY_VALUE',
'Maximum model space distance between geometric entities at asserted c
onnectivities');
#43467=(
GEOMETRIC_REPRESENTATION_CONTEXT(3)
GLOBAL_UNCERTAINTY_ASSIGNED_CONTEXT((#43399))
GLOBAL_UNIT_ASSIGNED_CONTEXT((#43522,#43524,#43525))
REPRESENTATION_CONTEXT('','3D')
);
#43521=(
GEOMETRIC_REPRESENTATION_CONTEXT(3)
GLOBAL_UNCERTAINTY_ASSIGNED_CONTEXT((#43453))
GLOBAL_UNIT_ASSIGNED_CONTEXT((#43522,#43524,#43525))
REPRESENTATION_CONTEXT('','3D')
);
#43522=(
LENGTH_UNIT()
NAMED_UNIT(*)
SI_UNIT(.CENTI.,.METRE.)
);
#43524=(
NAMED_UNIT(*)
PLANE_ANGLE_UNIT()
SI_UNIT($,.RADIAN.)
);
#43525=(
NAMED_UNIT(*)
SI_UNIT($,.STERADIAN.)
SOLID_ANGLE_UNIT()
);
#43539=SHAPE_DEFINITION_REPRESENTATION(#43606,#43807);
#43606=PRODUCT_DEFINITION_SHAPE('',$,#43875);
#43807=SHAPE_REPRESENTATION('',(#19613),#43467);
#43861=PRODUCT_DEFINITION_CONTEXT('part definition',#44064,'design');
#43875=PRODUCT_DEFINITION('Fixed bearing crossbar',
'Fixed bearing crossbar',#43942,#43861);
#43942=PRODUCT_DEFINITION_FORMATION('',$,#44079);
#44064=APPLICATION_CONTEXT(
'Core Data for Automotive Mechanical Design Process');
#44065=PRODUCT_CONTEXT('part definition',#44064,'mechanical');
#44079=PRODUCT('Fixed bearing crossbar','Fixed bearing crossbar',
'Fixed bearing crossbar',(#44065));
#44196=COLOUR_RGB('Grey',0.48,0.52,0.57);
#44197=FILL_AREA_STYLE_COLOUR('',#44196);
#44198=FILL_AREA_STYLE('',(#44197));
#44199=SURFACE_STYLE_FILL_AREA(#44198);
#44200=SURFACE_SIDE_STYLE('',(#44199));
#44201=SURFACE_STYLE_USAGE(.BOTH.,#44200);
#44202=PRESENTATION_STYLE_ASSIGNMENT((#44201));
ENDSEC;
END-ISO-10303-21;
